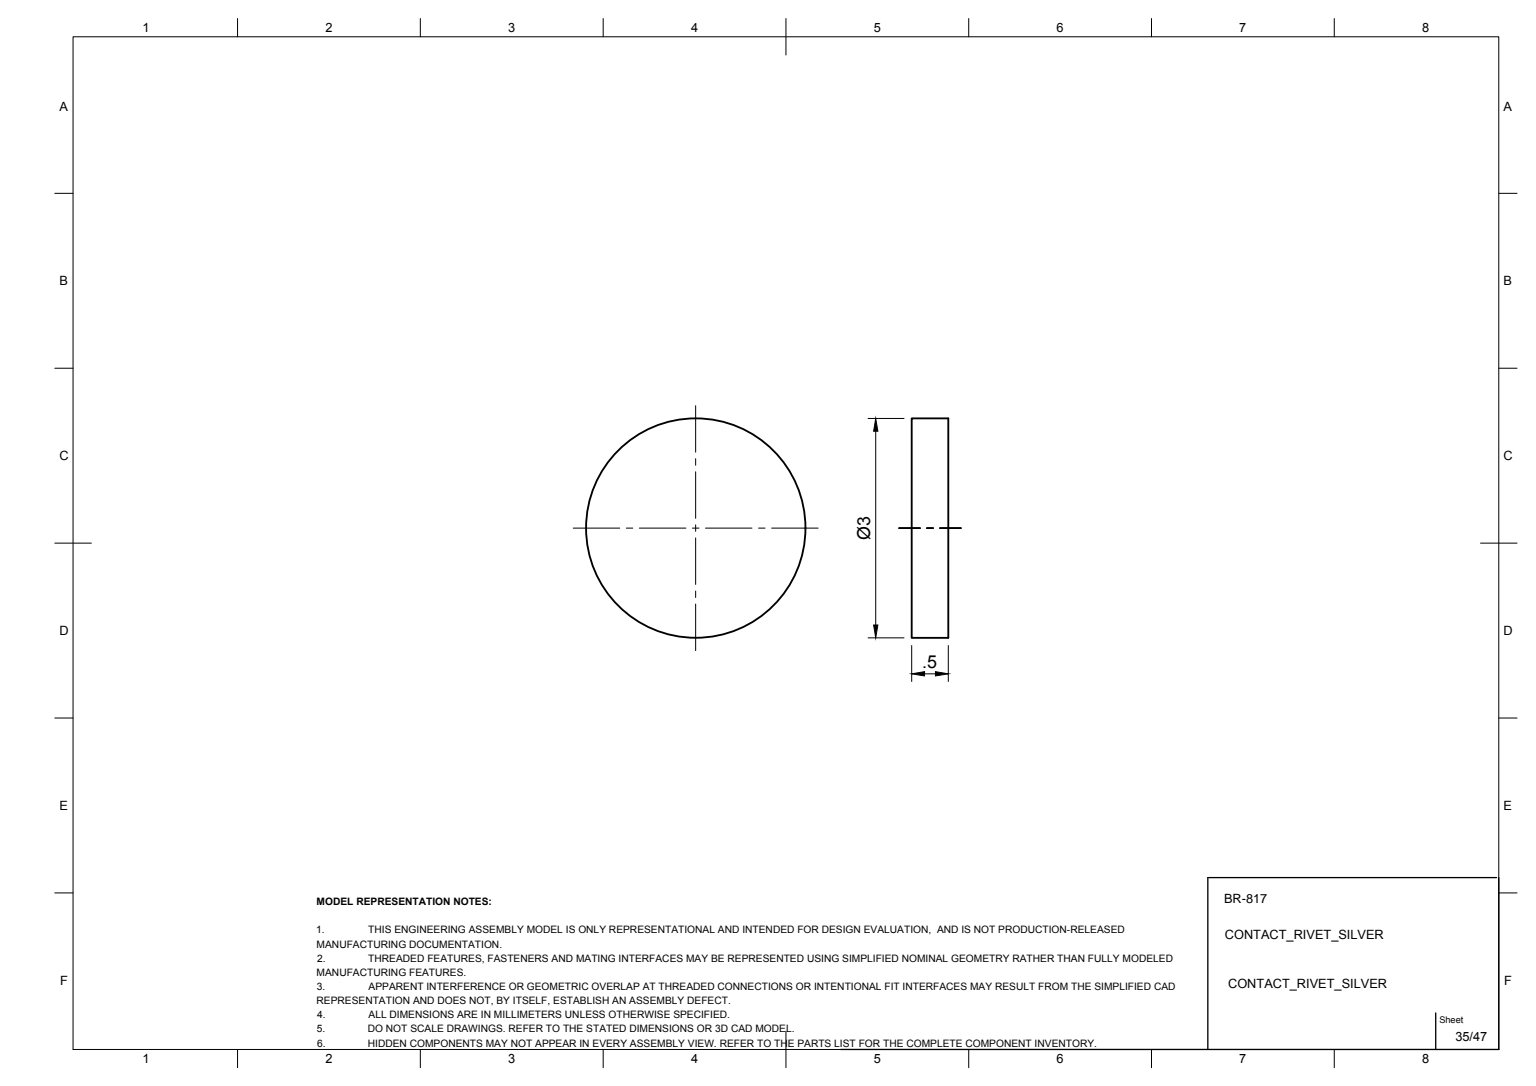
ISO-10303-21;
HEADER;
FILE_DESCRIPTION((''),'2;1');
FILE_NAME('CONTACT_RIVET_SILVER.step','2026-10-01T22:07:29-07:00',(''),(''),'','','');
FILE_SCHEMA (('AUTOMOTIVE_DESIGN { 1 0 10303 214 3 1 1 }'));
ENDSEC;
DATA;
#10=MECHANICAL_DESIGN_GEOMETRIC_PRESENTATION_REPRESENTATION('',(#568),#15484);
#497=SHAPE_REPRESENTATION_RELATIONSHIP('SRR','None',#15647,#532) ;
#532=ADVANCED_BREP_SHAPE_REPRESENTATION('',(#609),#15471) ;
#568=STYLED_ITEM('',(#15839),#609) ;
#609=MANIFOLD_SOLID_BREP('CONTACT_RIVET_SILVER',#8279) ;
#760=CYLINDRICAL_SURFACE('',#9543,0.15) ;
#1227=CIRCLE('',#9544,0.15) ;
#1228=CIRCLE('',#9545,0.15) ;
#1721=FACE_OUTER_BOUND('',#2287,.T.) ;
#1722=FACE_OUTER_BOUND('',#2288,.T.) ;
#1723=FACE_OUTER_BOUND('',#2289,.T.) ;
#2287=EDGE_LOOP('',(#6891,#6892,#6893,#6894)) ;
#2288=EDGE_LOOP('',(#6895)) ;
#2289=EDGE_LOOP('',(#6896)) ;
#2787=LINE('',#14680,#3261) ;
#3261=VECTOR('',#11998,0.15) ;
#3927=VERTEX_POINT('',#14677) ;
#3928=VERTEX_POINT('',#14679) ;
#4950=EDGE_CURVE('',#3927,#3927,#1227,.T.) ;
#4951=EDGE_CURVE('',#3927,#3928,#2787,.T.) ;
#4952=EDGE_CURVE('',#3928,#3928,#1228,.T.) ;
#6891=ORIENTED_EDGE('',*,*,#4950,.F.) ;
#6892=ORIENTED_EDGE('',*,*,#4951,.T.) ;
#6893=ORIENTED_EDGE('',*,*,#4952,.F.) ;
#6894=ORIENTED_EDGE('',*,*,#4951,.F.) ;
#6895=ORIENTED_EDGE('',*,*,#4952,.T.) ;
#6896=ORIENTED_EDGE('',*,*,#4950,.T.) ;
#7691=PLANE('',#9546) ;
#7692=PLANE('',#9547) ;
#8108=ADVANCED_FACE('',(#1721),#760,.T.) ;
#8109=ADVANCED_FACE('',(#1722),#7691,.T.) ;
#8110=ADVANCED_FACE('',(#1723),#7692,.T.) ;
#8279=CLOSED_SHELL('',(#8108,#8109,#8110)) ;
#9542=AXIS2_PLACEMENT_3D('',#14675,#11992,#11993) ;
#9543=AXIS2_PLACEMENT_3D('',#14676,#11994,#11995) ;
#9544=AXIS2_PLACEMENT_3D('',#14678,#11996,#11997) ;
#9545=AXIS2_PLACEMENT_3D('',#14681,#11999,#12000) ;
#9546=AXIS2_PLACEMENT_3D('',#14682,#12001,#12002) ;
#9547=AXIS2_PLACEMENT_3D('',#14683,#12003,#12004) ;
#11992=DIRECTION('axis',(0.,0.,1.)) ;
#11993=DIRECTION('refdir',(1.,0.,0.)) ;
#11994=DIRECTION('center_axis',(0.,0.,1.)) ;
#11995=DIRECTION('ref_axis',(1.,0.,0.)) ;
#11996=DIRECTION('center_axis',(0.,0.,1.)) ;
#11997=DIRECTION('ref_axis',(1.,0.,0.)) ;
#11998=DIRECTION('',(0.,0.,-1.)) ;
#11999=DIRECTION('center_axis',(0.,0.,-1.)) ;
#12000=DIRECTION('ref_axis',(1.,0.,0.)) ;
#12001=DIRECTION('center_axis',(0.,0.,-1.)) ;
#12002=DIRECTION('ref_axis',(-1.,0.,0.)) ;
#12003=DIRECTION('center_axis',(0.,0.,1.)) ;
#12004=DIRECTION('ref_axis',(1.,0.,0.)) ;
#14675=CARTESIAN_POINT('',(0.,0.,0.)) ;
#14676=CARTESIAN_POINT('Origin',(-1.1,-1.75,0.725)) ;
#14677=CARTESIAN_POINT('',(-1.25,-1.75,0.75)) ;
#14678=CARTESIAN_POINT('Origin',(-1.1,-1.75,0.75)) ;
#14679=CARTESIAN_POINT('',(-1.25,-1.75,0.7)) ;
#14680=CARTESIAN_POINT('',(-1.25,-1.75,0.725)) ;
#14681=CARTESIAN_POINT('Origin',(-1.1,-1.75,0.7)) ;
#14682=CARTESIAN_POINT('Origin',(-1.1,-1.75,0.7)) ;
#14683=CARTESIAN_POINT('Origin',(-1.1,-1.75,0.75)) ;
#15428=UNCERTAINTY_MEASURE_WITH_UNIT(LENGTH_MEASURE(0.001),#15485,
'DISTANCE_ACCURACY_VALUE',
'Maximum model space distance between geometric entities at asserted c
onnectivities') ;
#15441=UNCERTAINTY_MEASURE_WITH_UNIT(LENGTH_MEASURE(0.001),#15485,
'DISTANCE_ACCURACY_VALUE',
'Maximum model space distance between geometric entities at asserted c
onnectivities') ;
#15471=(
GEOMETRIC_REPRESENTATION_CONTEXT(3)
GLOBAL_UNCERTAINTY_ASSIGNED_CONTEXT((#15428))
GLOBAL_UNIT_ASSIGNED_CONTEXT((#15485,#15487,#15488))
REPRESENTATION_CONTEXT('','3D')
) ;
#15484=(
GEOMETRIC_REPRESENTATION_CONTEXT(3)
GLOBAL_UNCERTAINTY_ASSIGNED_CONTEXT((#15441))
GLOBAL_UNIT_ASSIGNED_CONTEXT((#15485,#15487,#15488))
REPRESENTATION_CONTEXT('','3D')
) ;
#15485=(
LENGTH_UNIT()
NAMED_UNIT(*)
SI_UNIT(.CENTI.,.METRE.)
) ;
#15487=(
NAMED_UNIT(*)
PLANE_ANGLE_UNIT()
SI_UNIT($,.RADIAN.)
) ;
#15488=(
NAMED_UNIT(*)
SI_UNIT($,.STERADIAN.)
SOLID_ANGLE_UNIT()
) ;
#15518=SHAPE_DEFINITION_REPRESENTATION(#15575,#15647) ;
#15575=PRODUCT_DEFINITION_SHAPE('',$,#15690) ;
#15647=SHAPE_REPRESENTATION('',(#9542),#15471) ;
#15660=PRODUCT_DEFINITION_CONTEXT('part definition',#15788,'design') ;
#15690=PRODUCT_DEFINITION('CONTACT_RIVET_SILVER',
'CONTACT_RIVET_SILVER',#15732,#15660) ;
#15732=PRODUCT_DEFINITION_FORMATION('',$,#15819) ;
#15788=APPLICATION_CONTEXT(
'Core Data for Automotive Mechanical Design Process') ;
#15789=PRODUCT_CONTEXT('part definition',#15788,'mechanical') ;
#15819=PRODUCT('CONTACT_RIVET_SILVER','CONTACT_RIVET_SILVER',$,(#15789)) ;
#15839=PRESENTATION_STYLE_ASSIGNMENT((#15851)) ;
#15851=SURFACE_STYLE_USAGE(.BOTH.,#15863) ;
#15863=SURFACE_SIDE_STYLE('',(#15875)) ;
#15875=SURFACE_STYLE_FILL_AREA(#15887) ;
#15887=FILL_AREA_STYLE('Nickel - Polished',(#15899)) ;
#15899=FILL_AREA_STYLE_COLOUR('Nickel - Polished',#15911) ;
#15911=COLOUR_RGB('Nickel - Polished', 0.31764706, 0.68627451, 0.89019608) ;
ENDSEC;
END-ISO-10303-21;
